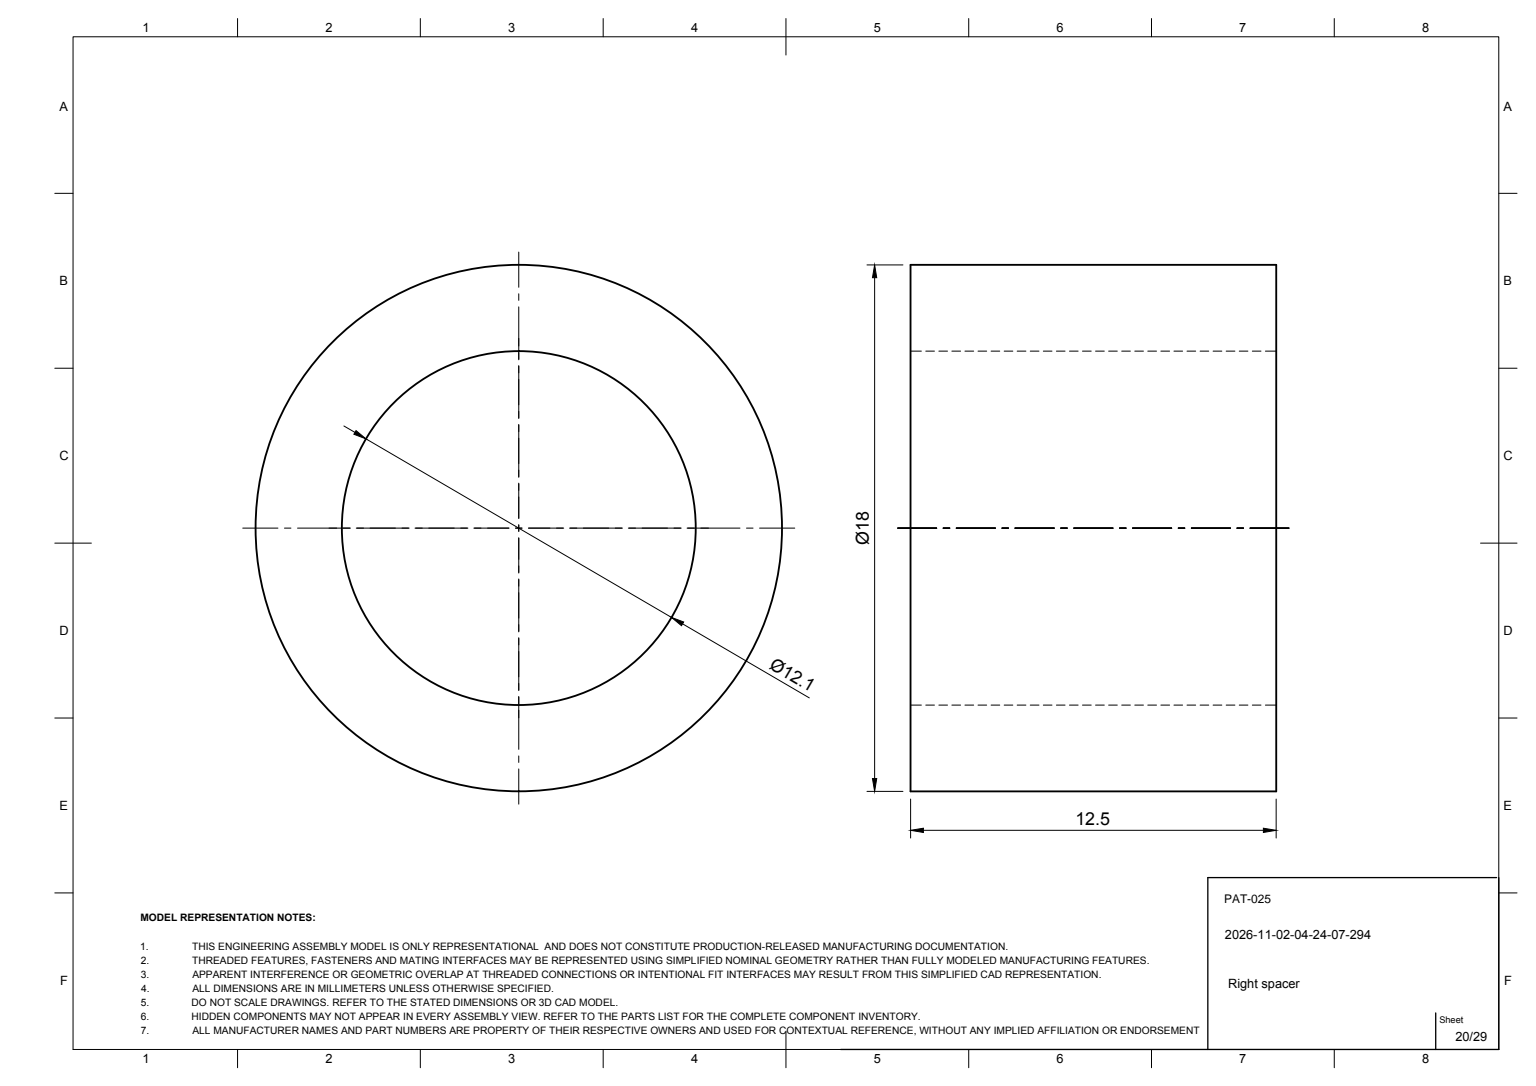
ISO-10303-21;
HEADER;
/* Generated by software containing ST-Developer
 * from STEP Tools, Inc. (www.steptools.com) 
 */

FILE_DESCRIPTION(
/* description */ ('Counter shaft with two pulleys and keyed hub'),
/* implementation_level */ '2;1');

FILE_NAME(
/* name */ 'Right spacer.step',
/* time_stamp */ '2026-10-27T10:46:10-07:00',
/* author */ (''),
/* organization */ (''),
/* preprocessor_version */ 'ST-DEVELOPER v20.2',
/* originating_system */ 'Autodesk Translation Framework v15.17.0.0',
/* authorisation */ '');

FILE_SCHEMA (('AUTOMOTIVE_DESIGN { 1 0 10303 214 3 1 1 }'));
ENDSEC;

DATA;
#10=MECHANICAL_DESIGN_GEOMETRIC_PRESENTATION_REPRESENTATION('',(#304),#10821);
#253=SHAPE_REPRESENTATION_RELATIONSHIP('SRR','None',#10941,#278);
#278=ADVANCED_BREP_SHAPE_REPRESENTATION('',(#329),#10809);
#304=STYLED_ITEM('',(#11121),#329);
#329=MANIFOLD_SOLID_BREP('Body1',#5588);
#397=FACE_BOUND('',#1091,.T.);
#398=FACE_BOUND('',#1093,.T.);
#517=PLANE('',#6130);
#518=PLANE('',#6131);
#717=FACE_OUTER_BOUND('',#1088,.T.);
#718=FACE_OUTER_BOUND('',#1089,.T.);
#719=FACE_OUTER_BOUND('',#1090,.T.);
#720=FACE_OUTER_BOUND('',#1092,.T.);
#1088=EDGE_LOOP('',(#4171,#4172,#4173,#4174));
#1089=EDGE_LOOP('',(#4175,#4176,#4177,#4178));
#1090=EDGE_LOOP('',(#4179));
#1091=EDGE_LOOP('',(#4180));
#1092=EDGE_LOOP('',(#4181));
#1093=EDGE_LOOP('',(#4182));
#1473=LINE('',#9348,#1862);
#1474=LINE('',#9354,#1863);
#1862=VECTOR('',#7223,0.605);
#1863=VECTOR('',#7230,0.9);
#2166=CIRCLE('',#6125,0.605);
#2167=CIRCLE('',#6126,0.605);
#2168=CIRCLE('',#6128,0.9);
#2169=CIRCLE('',#6129,0.9);
#2571=VERTEX_POINT('',#9345);
#2572=VERTEX_POINT('',#9347);
#2573=VERTEX_POINT('',#9351);
#2574=VERTEX_POINT('',#9353);
#3158=EDGE_CURVE('',#2571,#2571,#2166,.T.);
#3159=EDGE_CURVE('',#2571,#2572,#1473,.T.);
#3160=EDGE_CURVE('',#2572,#2572,#2167,.T.);
#3161=EDGE_CURVE('',#2573,#2573,#2168,.T.);
#3162=EDGE_CURVE('',#2573,#2574,#1474,.T.);
#3163=EDGE_CURVE('',#2574,#2574,#2169,.T.);
#4171=ORIENTED_EDGE('',*,*,#3158,.F.);
#4172=ORIENTED_EDGE('',*,*,#3159,.T.);
#4173=ORIENTED_EDGE('',*,*,#3160,.T.);
#4174=ORIENTED_EDGE('',*,*,#3159,.F.);
#4175=ORIENTED_EDGE('',*,*,#3161,.F.);
#4176=ORIENTED_EDGE('',*,*,#3162,.T.);
#4177=ORIENTED_EDGE('',*,*,#3163,.T.);
#4178=ORIENTED_EDGE('',*,*,#3162,.F.);
#4179=ORIENTED_EDGE('',*,*,#3161,.T.);
#4180=ORIENTED_EDGE('',*,*,#3158,.T.);
#4181=ORIENTED_EDGE('',*,*,#3163,.F.);
#4182=ORIENTED_EDGE('',*,*,#3160,.F.);
#5151=CYLINDRICAL_SURFACE('',#6124,0.605);
#5152=CYLINDRICAL_SURFACE('',#6127,0.9);
#5388=ADVANCED_FACE('',(#717),#5151,.F.);
#5389=ADVANCED_FACE('',(#718),#5152,.T.);
#5390=ADVANCED_FACE('',(#719,#397),#517,.T.);
#5391=ADVANCED_FACE('',(#720,#398),#518,.F.);
#5588=CLOSED_SHELL('',(#5388,#5389,#5390,#5391));
#6123=AXIS2_PLACEMENT_3D('',#9343,#7217,#7218);
#6124=AXIS2_PLACEMENT_3D('',#9344,#7219,#7220);
#6125=AXIS2_PLACEMENT_3D('',#9346,#7221,#7222);
#6126=AXIS2_PLACEMENT_3D('',#9349,#7224,#7225);
#6127=AXIS2_PLACEMENT_3D('',#9350,#7226,#7227);
#6128=AXIS2_PLACEMENT_3D('',#9352,#7228,#7229);
#6129=AXIS2_PLACEMENT_3D('',#9355,#7231,#7232);
#6130=AXIS2_PLACEMENT_3D('',#9356,#7233,#7234);
#6131=AXIS2_PLACEMENT_3D('',#9357,#7235,#7236);
#7217=DIRECTION('axis',(0.,0.,1.));
#7218=DIRECTION('refdir',(1.,0.,0.));
#7219=DIRECTION('center_axis',(0.,1.,0.));
#7220=DIRECTION('ref_axis',(1.,0.,0.));
#7221=DIRECTION('center_axis',(0.,-1.,0.));
#7222=DIRECTION('ref_axis',(1.,0.,0.));
#7223=DIRECTION('',(0.,-1.,0.));
#7224=DIRECTION('center_axis',(0.,-1.,0.));
#7225=DIRECTION('ref_axis',(1.,0.,0.));
#7226=DIRECTION('center_axis',(0.,1.,0.));
#7227=DIRECTION('ref_axis',(1.,0.,0.));
#7228=DIRECTION('center_axis',(0.,1.,0.));
#7229=DIRECTION('ref_axis',(1.,0.,0.));
#7230=DIRECTION('',(0.,-1.,0.));
#7231=DIRECTION('center_axis',(0.,1.,0.));
#7232=DIRECTION('ref_axis',(1.,0.,0.));
#7233=DIRECTION('center_axis',(0.,1.,0.));
#7234=DIRECTION('ref_axis',(1.,0.,0.));
#7235=DIRECTION('center_axis',(0.,1.,0.));
#7236=DIRECTION('ref_axis',(1.,0.,0.));
#9343=CARTESIAN_POINT('',(0.,0.,0.));
#9344=CARTESIAN_POINT('Origin',(0.,25.75,4.53));
#9345=CARTESIAN_POINT('',(-0.605,27.,4.53));
#9346=CARTESIAN_POINT('Origin',(0.,27.,4.53));
#9347=CARTESIAN_POINT('',(-0.605,25.75,4.53));
#9348=CARTESIAN_POINT('',(-0.605,25.75,4.53));
#9349=CARTESIAN_POINT('Origin',(0.,25.75,4.53));
#9350=CARTESIAN_POINT('Origin',(0.,25.75,4.53));
#9351=CARTESIAN_POINT('',(-0.9,27.,4.53));
#9352=CARTESIAN_POINT('Origin',(0.,27.,4.53));
#9353=CARTESIAN_POINT('',(-0.9,25.75,4.53));
#9354=CARTESIAN_POINT('',(-0.9,25.75,4.53));
#9355=CARTESIAN_POINT('Origin',(0.,25.75,4.53));
#9356=CARTESIAN_POINT('Origin',(0.,27.,4.53));
#9357=CARTESIAN_POINT('Origin',(0.,25.75,4.53));
#10779=UNCERTAINTY_MEASURE_WITH_UNIT(LENGTH_MEASURE(0.001),#10822,
'DISTANCE_ACCURACY_VALUE',
'Maximum model space distance between geometric entities at asserted c
onnectivities');
#10791=UNCERTAINTY_MEASURE_WITH_UNIT(LENGTH_MEASURE(0.001),#10822,
'DISTANCE_ACCURACY_VALUE',
'Maximum model space distance between geometric entities at asserted c
onnectivities');
#10809=(
GEOMETRIC_REPRESENTATION_CONTEXT(3)
GLOBAL_UNCERTAINTY_ASSIGNED_CONTEXT((#10779))
GLOBAL_UNIT_ASSIGNED_CONTEXT((#10822,#10824,#10825))
REPRESENTATION_CONTEXT('','3D')
);
#10821=(
GEOMETRIC_REPRESENTATION_CONTEXT(3)
GLOBAL_UNCERTAINTY_ASSIGNED_CONTEXT((#10791))
GLOBAL_UNIT_ASSIGNED_CONTEXT((#10822,#10824,#10825))
REPRESENTATION_CONTEXT('','3D')
);
#10822=(
LENGTH_UNIT()
NAMED_UNIT(*)
SI_UNIT(.CENTI.,.METRE.)
);
#10824=(
NAMED_UNIT(*)
PLANE_ANGLE_UNIT()
SI_UNIT($,.RADIAN.)
);
#10825=(
NAMED_UNIT(*)
SI_UNIT($,.STERADIAN.)
SOLID_ANGLE_UNIT()
);
#10843=SHAPE_DEFINITION_REPRESENTATION(#10891,#10941);
#10891=PRODUCT_DEFINITION_SHAPE('',$,#10971);
#10941=SHAPE_REPRESENTATION('',(#6123),#10809);
#10953=PRODUCT_DEFINITION_CONTEXT('part definition',#11042,'design');
#10971=PRODUCT_DEFINITION('Right spacer','Right spacer',#11000,#10953);
#11000=PRODUCT_DEFINITION_FORMATION('',$,#11061);
#11042=APPLICATION_CONTEXT(
'Core Data for Automotive Mechanical Design Process');
#11043=PRODUCT_CONTEXT('part definition',#11042,'mechanical');
#11061=PRODUCT('Right spacer','Right spacer','Right spacer',(#11043));
#11115=COLOUR_RGB('Light Blue',0.38,0.62,0.78);
#11116=FILL_AREA_STYLE_COLOUR('',#11115);
#11117=FILL_AREA_STYLE('',(#11116));
#11118=SURFACE_STYLE_FILL_AREA(#11117);
#11119=SURFACE_SIDE_STYLE('',(#11118));
#11120=SURFACE_STYLE_USAGE(.BOTH.,#11119);
#11121=PRESENTATION_STYLE_ASSIGNMENT((#11120));
ENDSEC;
END-ISO-10303-21;
